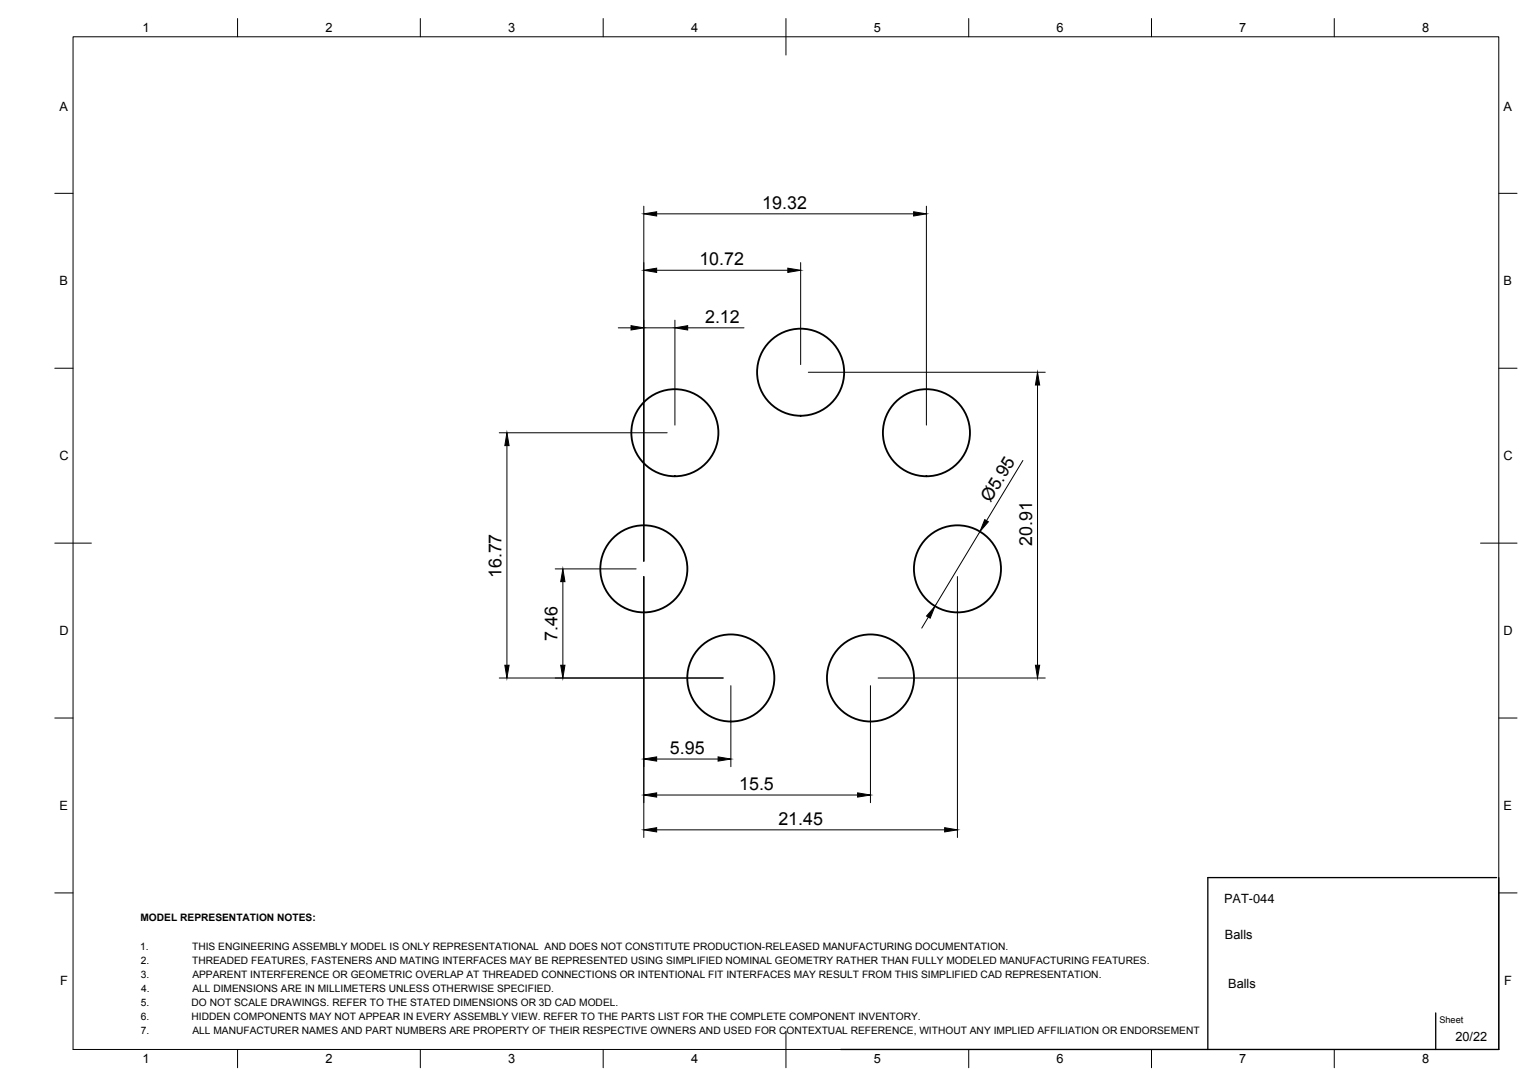
ISO-10303-21;
HEADER;
/* Generated by software containing ST-Developer
 * from STEP Tools, Inc. (www.steptools.com) 
 */

FILE_DESCRIPTION(
/* description */ ('Four-wheel beam trolley'),
/* implementation_level */ '2;1');

FILE_NAME(
/* name */ 'Balls.step',
/* time_stamp */ '2026-10-29T16:22:06-07:00',
/* author */ (''),
/* organization */ (''),
/* preprocessor_version */ 'ST-DEVELOPER v20.2',
/* originating_system */ 'Autodesk Translation Framework v15.17.0.0',
/* authorisation */ '');

FILE_SCHEMA (('AUTOMOTIVE_DESIGN { 1 0 10303 214 3 1 1 }'));
ENDSEC;

DATA;
#10=MECHANICAL_DESIGN_GEOMETRIC_PRESENTATION_REPRESENTATION('',(#291,#292,#293,#294,#295,#296,#297),#4777);
#25=SPHERICAL_SURFACE('',#2827,0.29765);
#26=SPHERICAL_SURFACE('',#2829,0.29765);
#27=SPHERICAL_SURFACE('',#2831,0.29765);
#28=SPHERICAL_SURFACE('',#2833,0.29765);
#29=SPHERICAL_SURFACE('',#2835,0.29765);
#30=SPHERICAL_SURFACE('',#2837,0.29765);
#31=SPHERICAL_SURFACE('',#2839,0.29765);
#257=SHAPE_REPRESENTATION_RELATIONSHIP('SRR','None',#4888,#274);
#274=ADVANCED_BREP_SHAPE_REPRESENTATION('',(#313,#314,#315,#316,#317,#318,
#319),#4773);
#291=STYLED_ITEM('',(#5056),#313);
#292=STYLED_ITEM('',(#5056),#314);
#293=STYLED_ITEM('',(#5056),#315);
#294=STYLED_ITEM('',(#5056),#316);
#295=STYLED_ITEM('',(#5056),#317);
#296=STYLED_ITEM('',(#5056),#318);
#297=STYLED_ITEM('',(#5056),#319);
#313=MANIFOLD_SOLID_BREP('Body1',#2380);
#314=MANIFOLD_SOLID_BREP('Body2',#2381);
#315=MANIFOLD_SOLID_BREP('Body3',#2382);
#316=MANIFOLD_SOLID_BREP('Body4',#2383);
#317=MANIFOLD_SOLID_BREP('Body5',#2384);
#318=MANIFOLD_SOLID_BREP('Body6',#2385);
#319=MANIFOLD_SOLID_BREP('Body7',#2386);
#553=FACE_OUTER_BOUND('',#734,.T.);
#554=FACE_OUTER_BOUND('',#735,.T.);
#555=FACE_OUTER_BOUND('',#736,.T.);
#556=FACE_OUTER_BOUND('',#737,.T.);
#557=FACE_OUTER_BOUND('',#738,.T.);
#558=FACE_OUTER_BOUND('',#739,.T.);
#559=FACE_OUTER_BOUND('',#740,.T.);
#734=EDGE_LOOP('',(#2029,#2030));
#735=EDGE_LOOP('',(#2031,#2032));
#736=EDGE_LOOP('',(#2033,#2034));
#737=EDGE_LOOP('',(#2035,#2036));
#738=EDGE_LOOP('',(#2037,#2038));
#739=EDGE_LOOP('',(#2039,#2040));
#740=EDGE_LOOP('',(#2041,#2042));
#1110=CIRCLE('',#2828,0.29765);
#1111=CIRCLE('',#2830,0.29765);
#1112=CIRCLE('',#2832,0.29765);
#1113=CIRCLE('',#2834,0.29765);
#1114=CIRCLE('',#2836,0.29765);
#1115=CIRCLE('',#2838,0.29765);
#1116=CIRCLE('',#2840,0.29765);
#1292=VERTEX_POINT('',#4256);
#1293=VERTEX_POINT('',#4257);
#1294=VERTEX_POINT('',#4260);
#1295=VERTEX_POINT('',#4261);
#1296=VERTEX_POINT('',#4264);
#1297=VERTEX_POINT('',#4265);
#1298=VERTEX_POINT('',#4268);
#1299=VERTEX_POINT('',#4269);
#1300=VERTEX_POINT('',#4272);
#1301=VERTEX_POINT('',#4273);
#1302=VERTEX_POINT('',#4276);
#1303=VERTEX_POINT('',#4277);
#1304=VERTEX_POINT('',#4280);
#1305=VERTEX_POINT('',#4281);
#1552=EDGE_CURVE('',#1292,#1293,#1110,.T.);
#1553=EDGE_CURVE('',#1294,#1295,#1111,.T.);
#1554=EDGE_CURVE('',#1296,#1297,#1112,.T.);
#1555=EDGE_CURVE('',#1298,#1299,#1113,.T.);
#1556=EDGE_CURVE('',#1300,#1301,#1114,.T.);
#1557=EDGE_CURVE('',#1302,#1303,#1115,.T.);
#1558=EDGE_CURVE('',#1304,#1305,#1116,.T.);
#2029=ORIENTED_EDGE('',*,*,#1552,.T.);
#2030=ORIENTED_EDGE('',*,*,#1552,.F.);
#2031=ORIENTED_EDGE('',*,*,#1553,.T.);
#2032=ORIENTED_EDGE('',*,*,#1553,.F.);
#2033=ORIENTED_EDGE('',*,*,#1554,.T.);
#2034=ORIENTED_EDGE('',*,*,#1554,.F.);
#2035=ORIENTED_EDGE('',*,*,#1555,.T.);
#2036=ORIENTED_EDGE('',*,*,#1555,.F.);
#2037=ORIENTED_EDGE('',*,*,#1556,.T.);
#2038=ORIENTED_EDGE('',*,*,#1556,.F.);
#2039=ORIENTED_EDGE('',*,*,#1557,.T.);
#2040=ORIENTED_EDGE('',*,*,#1557,.F.);
#2041=ORIENTED_EDGE('',*,*,#1558,.T.);
#2042=ORIENTED_EDGE('',*,*,#1558,.F.);
#2329=ADVANCED_FACE('',(#553),#25,.T.);
#2330=ADVANCED_FACE('',(#554),#26,.T.);
#2331=ADVANCED_FACE('',(#555),#27,.T.);
#2332=ADVANCED_FACE('',(#556),#28,.T.);
#2333=ADVANCED_FACE('',(#557),#29,.T.);
#2334=ADVANCED_FACE('',(#558),#30,.T.);
#2335=ADVANCED_FACE('',(#559),#31,.T.);
#2380=CLOSED_SHELL('',(#2329));
#2381=CLOSED_SHELL('',(#2330));
#2382=CLOSED_SHELL('',(#2331));
#2383=CLOSED_SHELL('',(#2332));
#2384=CLOSED_SHELL('',(#2333));
#2385=CLOSED_SHELL('',(#2334));
#2386=CLOSED_SHELL('',(#2335));
#2826=AXIS2_PLACEMENT_3D('',#4254,#3541,#3542);
#2827=AXIS2_PLACEMENT_3D('',#4255,#3543,#3544);
#2828=AXIS2_PLACEMENT_3D('',#4258,#3545,#3546);
#2829=AXIS2_PLACEMENT_3D('',#4259,#3547,#3548);
#2830=AXIS2_PLACEMENT_3D('',#4262,#3549,#3550);
#2831=AXIS2_PLACEMENT_3D('',#4263,#3551,#3552);
#2832=AXIS2_PLACEMENT_3D('',#4266,#3553,#3554);
#2833=AXIS2_PLACEMENT_3D('',#4267,#3555,#3556);
#2834=AXIS2_PLACEMENT_3D('',#4270,#3557,#3558);
#2835=AXIS2_PLACEMENT_3D('',#4271,#3559,#3560);
#2836=AXIS2_PLACEMENT_3D('',#4274,#3561,#3562);
#2837=AXIS2_PLACEMENT_3D('',#4275,#3563,#3564);
#2838=AXIS2_PLACEMENT_3D('',#4278,#3565,#3566);
#2839=AXIS2_PLACEMENT_3D('',#4279,#3567,#3568);
#2840=AXIS2_PLACEMENT_3D('',#4282,#3569,#3570);
#3541=DIRECTION('axis',(0.,0.,1.));
#3542=DIRECTION('refdir',(1.,0.,0.));
#3543=DIRECTION('center_axis',(0.,0.,1.));
#3544=DIRECTION('ref_axis',(1.,0.,0.));
#3545=DIRECTION('center_axis',(1.22464679914735E-16,-1.,0.));
#3546=DIRECTION('ref_axis',(-1.,-1.22464679914735E-16,0.));
#3547=DIRECTION('center_axis',(0.78183148246803,0.,0.623489801858733));
#3548=DIRECTION('ref_axis',(0.623489801858734,0.,-0.78183148246803));
#3549=DIRECTION('center_axis',(7.63554790147315E-17,-1.,-9.57467422477103E-17));
#3550=DIRECTION('ref_axis',(-0.623489801858734,-1.22464679914735E-16,0.78183148246803));
#3551=DIRECTION('center_axis',(0.974927912181824,0.,-0.222520933956314));
#3552=DIRECTION('ref_axis',(-0.222520933956314,0.,-0.974927912181824));
#3553=DIRECTION('center_axis',(-2.7250954951288E-17,-1.,-1.19394234705288E-16));
#3554=DIRECTION('ref_axis',(0.222520933956314,-1.22464679914735E-16,0.974927912181824));
#3555=DIRECTION('center_axis',(0.433883739117558,0.,-0.900968867902419));
#3556=DIRECTION('ref_axis',(-0.900968867902419,0.,-0.433883739117558));
#3557=DIRECTION('center_axis',(-1.10336864020811E-16,-1.,-5.31354332312403E-17));
#3558=DIRECTION('ref_axis',(0.900968867902419,-1.22464679914735E-16,0.433883739117558));
#3559=DIRECTION('center_axis',(-0.433883739117558,0.,-0.900968867902419));
#3560=DIRECTION('ref_axis',(-0.900968867902419,0.,0.433883739117558));
#3561=DIRECTION('center_axis',(-1.10336864020811E-16,-1.,5.31354332312403E-17));
#3562=DIRECTION('ref_axis',(0.900968867902419,-1.22464679914735E-16,-0.433883739117558));
#3563=DIRECTION('center_axis',(-0.974927912181824,0.,-0.222520933956314));
#3564=DIRECTION('ref_axis',(-0.222520933956315,0.,0.974927912181824));
#3565=DIRECTION('center_axis',(-2.7250954951288E-17,-1.,1.19394234705288E-16));
#3566=DIRECTION('ref_axis',(0.222520933956315,-1.22464679914735E-16,-0.974927912181824));
#3567=DIRECTION('center_axis',(-0.78183148246803,0.,0.623489801858734));
#3568=DIRECTION('ref_axis',(0.623489801858733,0.,0.78183148246803));
#3569=DIRECTION('center_axis',(7.63554790147315E-17,-1.,9.57467422477103E-17));
#3570=DIRECTION('ref_axis',(-0.623489801858733,-1.22464679914735E-16,-0.78183148246803));
#4254=CARTESIAN_POINT('',(0.,0.,0.));
#4255=CARTESIAN_POINT('Origin',(1.1,0.,0.));
#4256=CARTESIAN_POINT('',(1.1,-2.23201749654651E-33,0.29765));
#4257=CARTESIAN_POINT('',(1.1,-2.23201749654651E-33,-0.29765));
#4258=CARTESIAN_POINT('Origin',(1.1,0.,0.));
#4259=CARTESIAN_POINT('Origin',(0.685838782044607,0.,-0.860014630714833));
#4260=CARTESIAN_POINT('',(0.918550922801216,-5.31350540756609E-33,-0.674432891191581));
#4261=CARTESIAN_POINT('',(0.453126641287998,8.49470414473068E-34,-1.04559637023808));
#4262=CARTESIAN_POINT('Origin',(0.685838782044607,0.,-0.860014630714833));
#4263=CARTESIAN_POINT('Origin',(-0.244773027351946,0.,-1.07242070340001));
#4264=CARTESIAN_POINT('',(0.0454142657089739,-2.23201749654651E-33,-1.1386540593921));
#4265=CARTESIAN_POINT('',(-0.534960320412865,-2.23201749654651E-33,-1.00618734740791));
#4266=CARTESIAN_POINT('Origin',(-0.244773027351946,0.,-1.07242070340001));
#4267=CARTESIAN_POINT('Origin',(-0.991065754692661,0.,-0.477272113029314));
#4268=CARTESIAN_POINT('',(-0.86192025974432,8.49470414473067E-34,-0.745445496560469));
#4269=CARTESIAN_POINT('',(-1.120211249641,-5.31350540756609E-33,-0.209098729498159));
#4270=CARTESIAN_POINT('Origin',(-0.991065754692661,0.,-0.477272113029314));
#4271=CARTESIAN_POINT('Origin',(-0.991065754692661,0.,0.477272113029314));
#4272=CARTESIAN_POINT('',(-1.120211249641,-2.23201749654651E-33,0.209098729498159));
#4273=CARTESIAN_POINT('',(-0.86192025974432,-2.23201749654651E-33,0.745445496560469));
#4274=CARTESIAN_POINT('Origin',(-0.991065754692661,0.,0.477272113029314));
#4275=CARTESIAN_POINT('Origin',(-0.244773027351946,0.,1.07242070340001));
#4276=CARTESIAN_POINT('',(-0.534960320412866,-2.23201749654651E-33,1.00618734740791));
#4277=CARTESIAN_POINT('',(0.0454142657089737,-2.23201749654651E-33,1.1386540593921));
#4278=CARTESIAN_POINT('Origin',(-0.244773027351946,0.,1.07242070340001));
#4279=CARTESIAN_POINT('Origin',(0.685838782044607,0.,0.860014630714833));
#4280=CARTESIAN_POINT('',(0.453126641287998,-2.23201749654651E-33,1.04559637023808));
#4281=CARTESIAN_POINT('',(0.918550922801216,-2.23201749654651E-33,0.674432891191581));
#4282=CARTESIAN_POINT('Origin',(0.685838782044607,0.,0.860014630714833));
#4751=UNCERTAINTY_MEASURE_WITH_UNIT(LENGTH_MEASURE(0.001),#4778,
'DISTANCE_ACCURACY_VALUE',
'Maximum model space distance between geometric entities at asserted c
onnectivities');
#4755=UNCERTAINTY_MEASURE_WITH_UNIT(LENGTH_MEASURE(0.001),#4778,
'DISTANCE_ACCURACY_VALUE',
'Maximum model space distance between geometric entities at asserted c
onnectivities');
#4773=(
GEOMETRIC_REPRESENTATION_CONTEXT(3)
GLOBAL_UNCERTAINTY_ASSIGNED_CONTEXT((#4751))
GLOBAL_UNIT_ASSIGNED_CONTEXT((#4778,#4780,#4781))
REPRESENTATION_CONTEXT('','3D')
);
#4777=(
GEOMETRIC_REPRESENTATION_CONTEXT(3)
GLOBAL_UNCERTAINTY_ASSIGNED_CONTEXT((#4755))
GLOBAL_UNIT_ASSIGNED_CONTEXT((#4778,#4780,#4781))
REPRESENTATION_CONTEXT('','3D')
);
#4778=(
LENGTH_UNIT()
NAMED_UNIT(*)
SI_UNIT(.CENTI.,.METRE.)
);
#4780=(
NAMED_UNIT(*)
PLANE_ANGLE_UNIT()
SI_UNIT($,.RADIAN.)
);
#4781=(
NAMED_UNIT(*)
SI_UNIT($,.STERADIAN.)
SOLID_ANGLE_UNIT()
);
#4799=SHAPE_DEFINITION_REPRESENTATION(#4852,#4888);
#4852=PRODUCT_DEFINITION_SHAPE('',$,#4910);
#4888=SHAPE_REPRESENTATION('',(#2826),#4773);
#4892=PRODUCT_DEFINITION_CONTEXT('part definition',#4957,'design');
#4910=PRODUCT_DEFINITION('Balls','Balls',#4931,#4892);
#4931=PRODUCT_DEFINITION_FORMATION('',$,#4976);
#4957=APPLICATION_CONTEXT(
'Core Data for Automotive Mechanical Design Process');
#4958=PRODUCT_CONTEXT('part definition',#4957,'mechanical');
#4976=PRODUCT('Balls','Balls','Balls',(#4958));
#5050=COLOUR_RGB('Grey',0.48,0.52,0.57);
#5051=FILL_AREA_STYLE_COLOUR('',#5050);
#5052=FILL_AREA_STYLE('',(#5051));
#5053=SURFACE_STYLE_FILL_AREA(#5052);
#5054=SURFACE_SIDE_STYLE('',(#5053));
#5055=SURFACE_STYLE_USAGE(.BOTH.,#5054);
#5056=PRESENTATION_STYLE_ASSIGNMENT((#5055));
ENDSEC;
END-ISO-10303-21;
